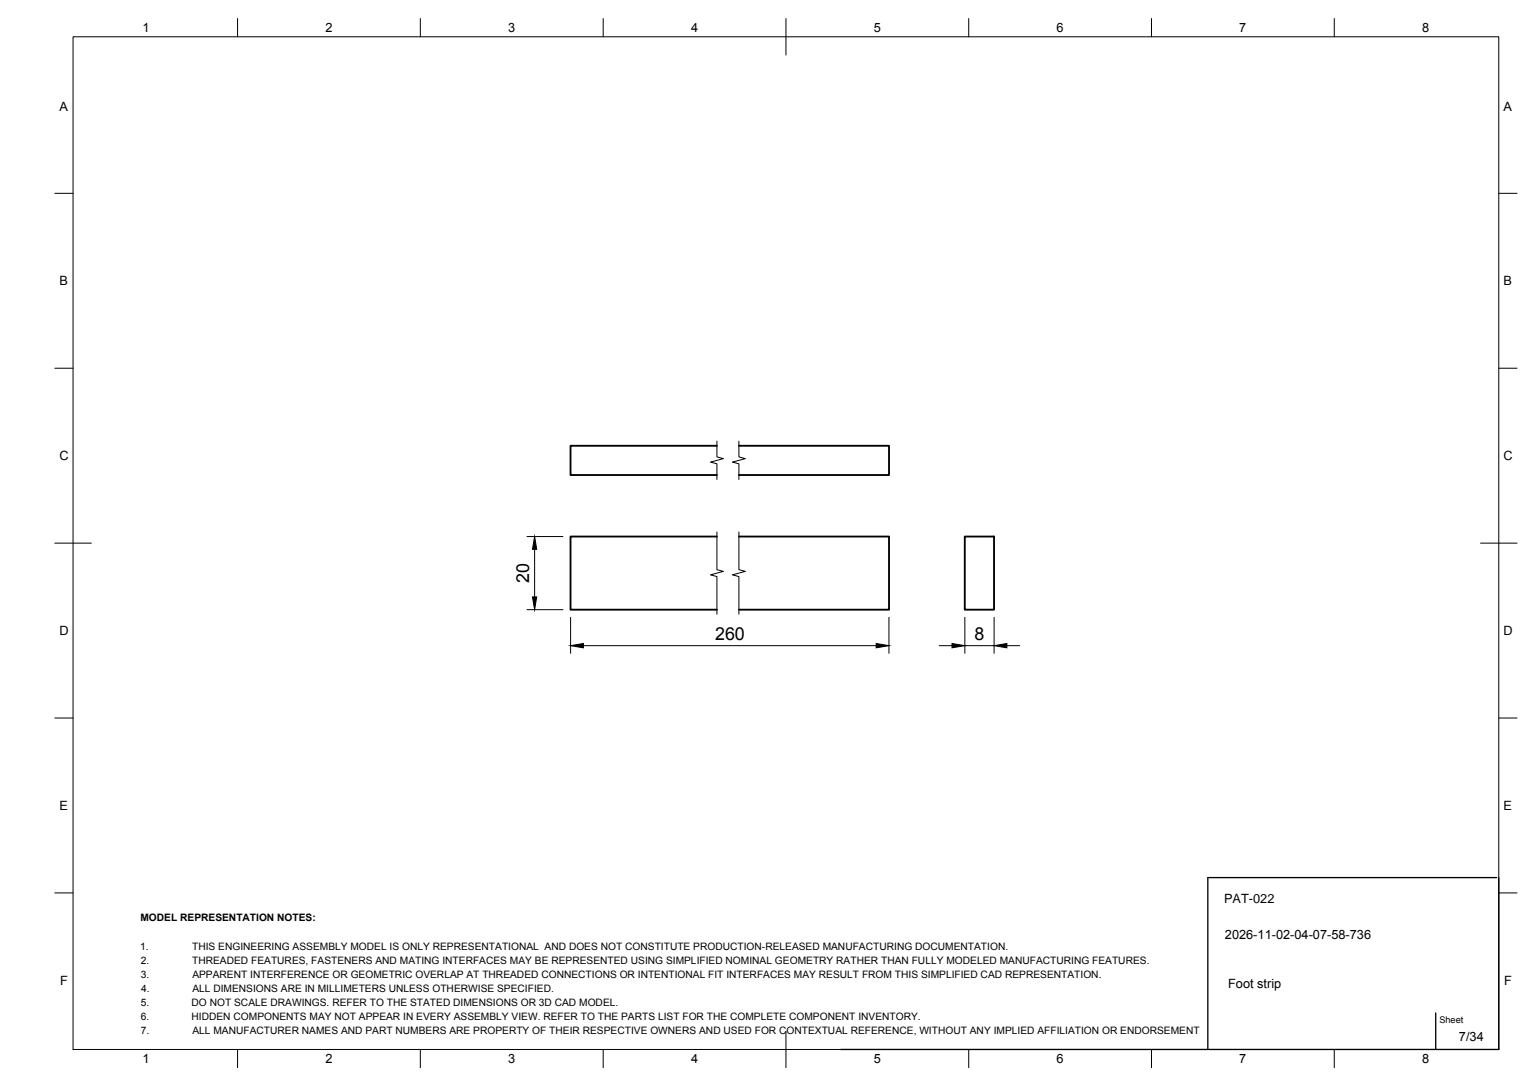
ISO-10303-21;
HEADER;
/* Generated by software containing ST-Developer
 * from STEP Tools, Inc. (www.steptools.com) 
 */

FILE_DESCRIPTION(
/* description */ ('Chute with adjustable gate'),
/* implementation_level */ '2;1');

FILE_NAME(
/* name */ 'Foot strip.step',
/* time_stamp */ '2026-10-27T10:52:28-07:00',
/* author */ (''),
/* organization */ (''),
/* preprocessor_version */ 'ST-DEVELOPER v20.2',
/* originating_system */ 'Autodesk Translation Framework v15.17.0.0',
/* authorisation */ '');

FILE_SCHEMA (('AUTOMOTIVE_DESIGN { 1 0 10303 214 3 1 1 }'));
ENDSEC;

DATA;
#10=MECHANICAL_DESIGN_GEOMETRIC_PRESENTATION_REPRESENTATION('',(#416),#13094);
#352=SHAPE_REPRESENTATION_RELATIONSHIP('SRR','None',#13253,#384);
#384=ADVANCED_BREP_SHAPE_REPRESENTATION('',(#448),#13062);
#416=STYLED_ITEM('',(#13481),#448);
#448=MANIFOLD_SOLID_BREP('Body1',#7599);
#606=PLANE('',#8031);
#607=PLANE('',#8032);
#608=PLANE('',#8033);
#609=PLANE('',#8034);
#610=PLANE('',#8035);
#611=PLANE('',#8036);
#938=FACE_OUTER_BOUND('',#1371,.T.);
#939=FACE_OUTER_BOUND('',#1372,.T.);
#940=FACE_OUTER_BOUND('',#1373,.T.);
#941=FACE_OUTER_BOUND('',#1374,.T.);
#942=FACE_OUTER_BOUND('',#1375,.T.);
#943=FACE_OUTER_BOUND('',#1376,.T.);
#1371=EDGE_LOOP('',(#5306,#5307,#5308,#5309));
#1372=EDGE_LOOP('',(#5310,#5311,#5312,#5313));
#1373=EDGE_LOOP('',(#5314,#5315,#5316,#5317));
#1374=EDGE_LOOP('',(#5318,#5319,#5320,#5321));
#1375=EDGE_LOOP('',(#5322,#5323,#5324,#5325));
#1376=EDGE_LOOP('',(#5326,#5327,#5328,#5329));
#1904=LINE('',#11031,#2681);
#1905=LINE('',#11033,#2682);
#1906=LINE('',#11035,#2683);
#1907=LINE('',#11036,#2684);
#1908=LINE('',#11039,#2685);
#1909=LINE('',#11041,#2686);
#1910=LINE('',#11042,#2687);
#1911=LINE('',#11045,#2688);
#1912=LINE('',#11047,#2689);
#1913=LINE('',#11048,#2690);
#1914=LINE('',#11050,#2691);
#1915=LINE('',#11051,#2692);
#2681=VECTOR('',#8834,1.);
#2682=VECTOR('',#8835,1.);
#2683=VECTOR('',#8836,1.);
#2684=VECTOR('',#8837,1.);
#2685=VECTOR('',#8840,1.);
#2686=VECTOR('',#8841,1.);
#2687=VECTOR('',#8842,1.);
#2688=VECTOR('',#8845,1.);
#2689=VECTOR('',#8846,1.);
#2690=VECTOR('',#8847,1.);
#2691=VECTOR('',#8850,1.);
#2692=VECTOR('',#8851,1.);
#3633=VERTEX_POINT('',#11029);
#3634=VERTEX_POINT('',#11030);
#3635=VERTEX_POINT('',#11032);
#3636=VERTEX_POINT('',#11034);
#3637=VERTEX_POINT('',#11038);
#3638=VERTEX_POINT('',#11040);
#3639=VERTEX_POINT('',#11044);
#3640=VERTEX_POINT('',#11046);
#4286=EDGE_CURVE('',#3633,#3634,#1904,.T.);
#4287=EDGE_CURVE('',#3634,#3635,#1905,.T.);
#4288=EDGE_CURVE('',#3636,#3635,#1906,.T.);
#4289=EDGE_CURVE('',#3633,#3636,#1907,.T.);
#4290=EDGE_CURVE('',#3637,#3633,#1908,.T.);
#4291=EDGE_CURVE('',#3638,#3636,#1909,.T.);
#4292=EDGE_CURVE('',#3637,#3638,#1910,.T.);
#4293=EDGE_CURVE('',#3639,#3637,#1911,.T.);
#4294=EDGE_CURVE('',#3640,#3638,#1912,.T.);
#4295=EDGE_CURVE('',#3639,#3640,#1913,.T.);
#4296=EDGE_CURVE('',#3634,#3639,#1914,.T.);
#4297=EDGE_CURVE('',#3635,#3640,#1915,.T.);
#5306=ORIENTED_EDGE('',*,*,#4286,.T.);
#5307=ORIENTED_EDGE('',*,*,#4287,.T.);
#5308=ORIENTED_EDGE('',*,*,#4288,.F.);
#5309=ORIENTED_EDGE('',*,*,#4289,.F.);
#5310=ORIENTED_EDGE('',*,*,#4290,.T.);
#5311=ORIENTED_EDGE('',*,*,#4289,.T.);
#5312=ORIENTED_EDGE('',*,*,#4291,.F.);
#5313=ORIENTED_EDGE('',*,*,#4292,.F.);
#5314=ORIENTED_EDGE('',*,*,#4293,.T.);
#5315=ORIENTED_EDGE('',*,*,#4292,.T.);
#5316=ORIENTED_EDGE('',*,*,#4294,.F.);
#5317=ORIENTED_EDGE('',*,*,#4295,.F.);
#5318=ORIENTED_EDGE('',*,*,#4296,.T.);
#5319=ORIENTED_EDGE('',*,*,#4295,.T.);
#5320=ORIENTED_EDGE('',*,*,#4297,.F.);
#5321=ORIENTED_EDGE('',*,*,#4287,.F.);
#5322=ORIENTED_EDGE('',*,*,#4297,.T.);
#5323=ORIENTED_EDGE('',*,*,#4294,.T.);
#5324=ORIENTED_EDGE('',*,*,#4291,.T.);
#5325=ORIENTED_EDGE('',*,*,#4288,.T.);
#5326=ORIENTED_EDGE('',*,*,#4296,.F.);
#5327=ORIENTED_EDGE('',*,*,#4286,.F.);
#5328=ORIENTED_EDGE('',*,*,#4290,.F.);
#5329=ORIENTED_EDGE('',*,*,#4293,.F.);
#7206=ADVANCED_FACE('',(#938),#606,.T.);
#7207=ADVANCED_FACE('',(#939),#607,.T.);
#7208=ADVANCED_FACE('',(#940),#608,.T.);
#7209=ADVANCED_FACE('',(#941),#609,.T.);
#7210=ADVANCED_FACE('',(#942),#610,.T.);
#7211=ADVANCED_FACE('',(#943),#611,.F.);
#7599=CLOSED_SHELL('',(#7206,#7207,#7208,#7209,#7210,#7211));
#8030=AXIS2_PLACEMENT_3D('',#11027,#8830,#8831);
#8031=AXIS2_PLACEMENT_3D('',#11028,#8832,#8833);
#8032=AXIS2_PLACEMENT_3D('',#11037,#8838,#8839);
#8033=AXIS2_PLACEMENT_3D('',#11043,#8843,#8844);
#8034=AXIS2_PLACEMENT_3D('',#11049,#8848,#8849);
#8035=AXIS2_PLACEMENT_3D('',#11052,#8852,#8853);
#8036=AXIS2_PLACEMENT_3D('',#11053,#8854,#8855);
#8830=DIRECTION('axis',(0.,0.,1.));
#8831=DIRECTION('refdir',(1.,0.,0.));
#8832=DIRECTION('center_axis',(0.,1.,0.));
#8833=DIRECTION('ref_axis',(-1.,0.,0.));
#8834=DIRECTION('',(-1.,0.,0.));
#8835=DIRECTION('',(0.,0.,1.));
#8836=DIRECTION('',(-1.,0.,0.));
#8837=DIRECTION('',(0.,0.,1.));
#8838=DIRECTION('center_axis',(1.,0.,0.));
#8839=DIRECTION('ref_axis',(0.,1.,0.));
#8840=DIRECTION('',(0.,1.,0.));
#8841=DIRECTION('',(0.,1.,0.));
#8842=DIRECTION('',(0.,0.,1.));
#8843=DIRECTION('center_axis',(0.,-1.,0.));
#8844=DIRECTION('ref_axis',(1.,0.,0.));
#8845=DIRECTION('',(1.,0.,0.));
#8846=DIRECTION('',(1.,0.,0.));
#8847=DIRECTION('',(0.,0.,1.));
#8848=DIRECTION('center_axis',(-1.,0.,0.));
#8849=DIRECTION('ref_axis',(0.,-1.,0.));
#8850=DIRECTION('',(0.,-1.,0.));
#8851=DIRECTION('',(0.,-1.,0.));
#8852=DIRECTION('center_axis',(0.,0.,1.));
#8853=DIRECTION('ref_axis',(1.,0.,0.));
#8854=DIRECTION('center_axis',(0.,0.,1.));
#8855=DIRECTION('ref_axis',(1.,0.,0.));
#11027=CARTESIAN_POINT('',(0.,0.,0.));
#11028=CARTESIAN_POINT('Origin',(2.,13.,-1.8));
#11029=CARTESIAN_POINT('',(2.,13.,-1.8));
#11030=CARTESIAN_POINT('',(0.,13.,-1.8));
#11031=CARTESIAN_POINT('',(2.,13.,-1.8));
#11032=CARTESIAN_POINT('',(0.,13.,-1.));
#11033=CARTESIAN_POINT('',(0.,13.,-1.8));
#11034=CARTESIAN_POINT('',(2.,13.,-1.));
#11035=CARTESIAN_POINT('',(2.,13.,-1.));
#11036=CARTESIAN_POINT('',(2.,13.,-1.8));
#11037=CARTESIAN_POINT('Origin',(2.,-13.,-1.8));
#11038=CARTESIAN_POINT('',(2.,-13.,-1.8));
#11039=CARTESIAN_POINT('',(2.,-13.,-1.8));
#11040=CARTESIAN_POINT('',(2.,-13.,-1.));
#11041=CARTESIAN_POINT('',(2.,-13.,-1.));
#11042=CARTESIAN_POINT('',(2.,-13.,-1.8));
#11043=CARTESIAN_POINT('Origin',(0.,-13.,-1.8));
#11044=CARTESIAN_POINT('',(0.,-13.,-1.8));
#11045=CARTESIAN_POINT('',(0.,-13.,-1.8));
#11046=CARTESIAN_POINT('',(0.,-13.,-1.));
#11047=CARTESIAN_POINT('',(0.,-13.,-1.));
#11048=CARTESIAN_POINT('',(0.,-13.,-1.8));
#11049=CARTESIAN_POINT('Origin',(0.,13.,-1.8));
#11050=CARTESIAN_POINT('',(0.,13.,-1.8));
#11051=CARTESIAN_POINT('',(0.,13.,-1.));
#11052=CARTESIAN_POINT('Origin',(1.,0.,-1.));
#11053=CARTESIAN_POINT('Origin',(1.,0.,-1.8));
#13025=UNCERTAINTY_MEASURE_WITH_UNIT(LENGTH_MEASURE(0.001),#13095,
'DISTANCE_ACCURACY_VALUE',
'Maximum model space distance between geometric entities at asserted c
onnectivities');
#13057=UNCERTAINTY_MEASURE_WITH_UNIT(LENGTH_MEASURE(0.001),#13095,
'DISTANCE_ACCURACY_VALUE',
'Maximum model space distance between geometric entities at asserted c
onnectivities');
#13062=(
GEOMETRIC_REPRESENTATION_CONTEXT(3)
GLOBAL_UNCERTAINTY_ASSIGNED_CONTEXT((#13025))
GLOBAL_UNIT_ASSIGNED_CONTEXT((#13095,#13097,#13098))
REPRESENTATION_CONTEXT('','3D')
);
#13094=(
GEOMETRIC_REPRESENTATION_CONTEXT(3)
GLOBAL_UNCERTAINTY_ASSIGNED_CONTEXT((#13057))
GLOBAL_UNIT_ASSIGNED_CONTEXT((#13095,#13097,#13098))
REPRESENTATION_CONTEXT('','3D')
);
#13095=(
LENGTH_UNIT()
NAMED_UNIT(*)
SI_UNIT(.CENTI.,.METRE.)
);
#13097=(
NAMED_UNIT(*)
PLANE_ANGLE_UNIT()
SI_UNIT($,.RADIAN.)
);
#13098=(
NAMED_UNIT(*)
SI_UNIT($,.STERADIAN.)
SOLID_ANGLE_UNIT()
);
#13103=SHAPE_DEFINITION_REPRESENTATION(#13139,#13253);
#13139=PRODUCT_DEFINITION_SHAPE('',$,#13290);
#13253=SHAPE_REPRESENTATION('',(#8030),#13062);
#13285=PRODUCT_DEFINITION_CONTEXT('part definition',#13395,'design');
#13290=PRODUCT_DEFINITION('Foot strip','Foot strip',#13326,#13285);
#13326=PRODUCT_DEFINITION_FORMATION('',$,#13401);
#13395=APPLICATION_CONTEXT(
'Core Data for Automotive Mechanical Design Process');
#13396=PRODUCT_CONTEXT('part definition',#13395,'mechanical');
#13401=PRODUCT('Foot strip','Foot strip','Foot strip',(#13396));
#13475=COLOUR_RGB('Light Blue',0.38,0.62,0.78);
#13476=FILL_AREA_STYLE_COLOUR('',#13475);
#13477=FILL_AREA_STYLE('',(#13476));
#13478=SURFACE_STYLE_FILL_AREA(#13477);
#13479=SURFACE_SIDE_STYLE('',(#13478));
#13480=SURFACE_STYLE_USAGE(.BOTH.,#13479);
#13481=PRESENTATION_STYLE_ASSIGNMENT((#13480));
ENDSEC;
END-ISO-10303-21;
